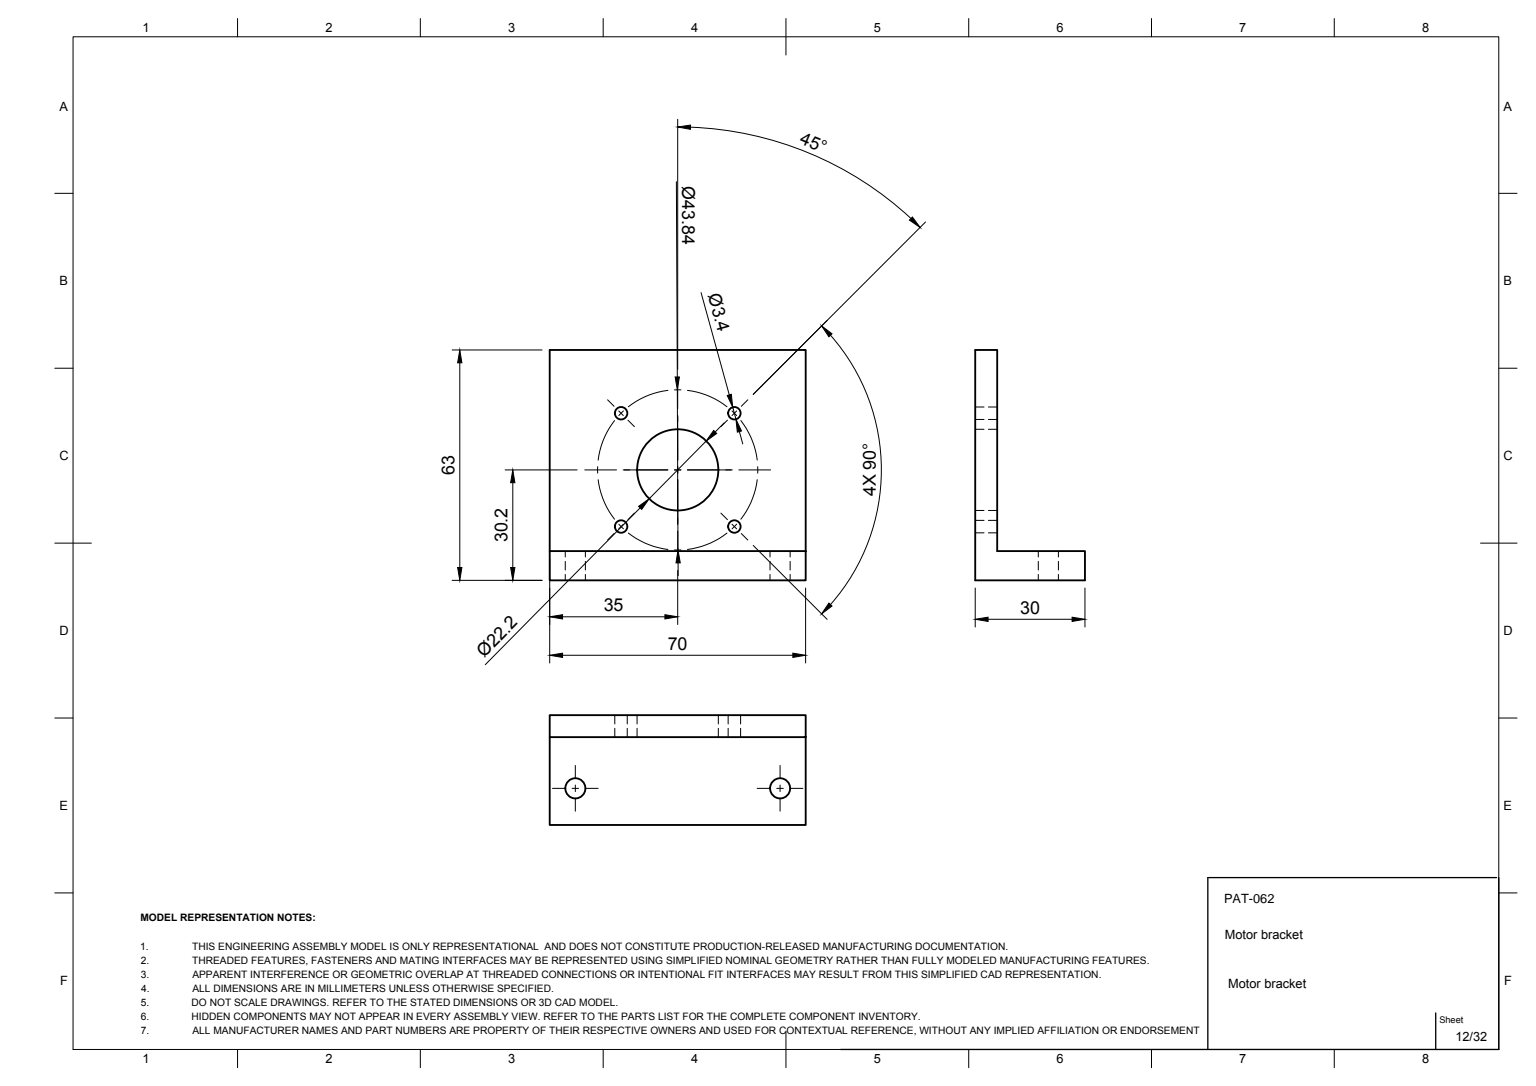
ISO-10303-21;
HEADER;
/* Generated by software containing ST-Developer
 * from STEP Tools, Inc. (www.steptools.com) 
 */

FILE_DESCRIPTION(
/* description */ ('Jaw-coupled motor to shaft test stand'),
/* implementation_level */ '2;1');

FILE_NAME(
/* name */ 'Motor bracket.step',
/* time_stamp */ '2026-10-27T10:46:06-07:00',
/* author */ (''),
/* organization */ (''),
/* preprocessor_version */ 'ST-DEVELOPER v20.2',
/* originating_system */ 'Autodesk Translation Framework v15.17.0.0',
/* authorisation */ '');

FILE_SCHEMA (('AUTOMOTIVE_DESIGN { 1 0 10303 214 3 1 1 }'));
ENDSEC;

DATA;
#10=MECHANICAL_DESIGN_GEOMETRIC_PRESENTATION_REPRESENTATION('',(#347),#19361);
#283=SHAPE_REPRESENTATION_RELATIONSHIP('SRR','None',#19497,#315);
#315=ADVANCED_BREP_SHAPE_REPRESENTATION('',(#380),#19333);
#347=STYLED_ITEM('',(#19725),#380);
#380=MANIFOLD_SOLID_BREP('Body1',#10991);
#423=FACE_BOUND('',#1710,.T.);
#424=FACE_BOUND('',#1711,.T.);
#425=FACE_BOUND('',#1714,.T.);
#426=FACE_BOUND('',#1715,.T.);
#427=FACE_BOUND('',#1716,.T.);
#428=FACE_BOUND('',#1717,.T.);
#429=FACE_BOUND('',#1718,.T.);
#430=FACE_BOUND('',#1722,.T.);
#431=FACE_BOUND('',#1723,.T.);
#432=FACE_BOUND('',#1724,.T.);
#433=FACE_BOUND('',#1725,.T.);
#434=FACE_BOUND('',#1726,.T.);
#435=FACE_BOUND('',#1729,.T.);
#436=FACE_BOUND('',#1730,.T.);
#542=PLANE('',#11472);
#543=PLANE('',#11473);
#544=PLANE('',#11474);
#545=PLANE('',#11475);
#546=PLANE('',#11476);
#547=PLANE('',#11477);
#548=PLANE('',#11478);
#549=PLANE('',#11479);
#1062=FACE_OUTER_BOUND('',#1702,.T.);
#1063=FACE_OUTER_BOUND('',#1703,.T.);
#1064=FACE_OUTER_BOUND('',#1704,.T.);
#1065=FACE_OUTER_BOUND('',#1705,.T.);
#1066=FACE_OUTER_BOUND('',#1706,.T.);
#1067=FACE_OUTER_BOUND('',#1707,.T.);
#1068=FACE_OUTER_BOUND('',#1708,.T.);
#1069=FACE_OUTER_BOUND('',#1709,.T.);
#1070=FACE_OUTER_BOUND('',#1712,.T.);
#1071=FACE_OUTER_BOUND('',#1713,.T.);
#1072=FACE_OUTER_BOUND('',#1719,.T.);
#1073=FACE_OUTER_BOUND('',#1720,.T.);
#1074=FACE_OUTER_BOUND('',#1721,.T.);
#1075=FACE_OUTER_BOUND('',#1727,.T.);
#1076=FACE_OUTER_BOUND('',#1728,.T.);
#1702=EDGE_LOOP('',(#7502,#7503,#7504,#7505));
#1703=EDGE_LOOP('',(#7506,#7507,#7508,#7509));
#1704=EDGE_LOOP('',(#7510,#7511,#7512,#7513));
#1705=EDGE_LOOP('',(#7514,#7515,#7516,#7517));
#1706=EDGE_LOOP('',(#7518,#7519,#7520,#7521));
#1707=EDGE_LOOP('',(#7522,#7523,#7524,#7525));
#1708=EDGE_LOOP('',(#7526,#7527,#7528,#7529));
#1709=EDGE_LOOP('',(#7530,#7531,#7532,#7533));
#1710=EDGE_LOOP('',(#7534));
#1711=EDGE_LOOP('',(#7535));
#1712=EDGE_LOOP('',(#7536,#7537,#7538,#7539));
#1713=EDGE_LOOP('',(#7540,#7541,#7542,#7543));
#1714=EDGE_LOOP('',(#7544));
#1715=EDGE_LOOP('',(#7545));
#1716=EDGE_LOOP('',(#7546));
#1717=EDGE_LOOP('',(#7547));
#1718=EDGE_LOOP('',(#7548));
#1719=EDGE_LOOP('',(#7549,#7550,#7551,#7552,#7553,#7554));
#1720=EDGE_LOOP('',(#7555,#7556,#7557,#7558,#7559,#7560));
#1721=EDGE_LOOP('',(#7561,#7562,#7563,#7564));
#1722=EDGE_LOOP('',(#7565));
#1723=EDGE_LOOP('',(#7566));
#1724=EDGE_LOOP('',(#7567));
#1725=EDGE_LOOP('',(#7568));
#1726=EDGE_LOOP('',(#7569));
#1727=EDGE_LOOP('',(#7570,#7571,#7572,#7573));
#1728=EDGE_LOOP('',(#7574,#7575,#7576,#7577));
#1729=EDGE_LOOP('',(#7578));
#1730=EDGE_LOOP('',(#7579));
#2425=LINE('',#15611,#3578);
#2426=LINE('',#15617,#3579);
#2427=LINE('',#15623,#3580);
#2428=LINE('',#15629,#3581);
#2429=LINE('',#15635,#3582);
#2430=LINE('',#15641,#3583);
#2431=LINE('',#15647,#3584);
#2432=LINE('',#15652,#3585);
#2433=LINE('',#15654,#3586);
#2434=LINE('',#15656,#3587);
#2435=LINE('',#15657,#3588);
#2436=LINE('',#15660,#3589);
#2437=LINE('',#15662,#3590);
#2438=LINE('',#15663,#3591);
#2439=LINE('',#15667,#3592);
#2440=LINE('',#15669,#3593);
#2441=LINE('',#15671,#3594);
#2442=LINE('',#15672,#3595);
#2443=LINE('',#15675,#3596);
#2444=LINE('',#15676,#3597);
#2445=LINE('',#15677,#3598);
#2446=LINE('',#15680,#3599);
#2447=LINE('',#15681,#3600);
#2448=LINE('',#15682,#3601);
#2449=LINE('',#15684,#3602);
#3578=VECTOR('',#12550,0.17);
#3579=VECTOR('',#12557,0.17);
#3580=VECTOR('',#12564,0.17);
#3581=VECTOR('',#12571,0.17);
#3582=VECTOR('',#12578,1.11);
#3583=VECTOR('',#12585,0.275);
#3584=VECTOR('',#12592,0.275);
#3585=VECTOR('',#12597,1.);
#3586=VECTOR('',#12598,1.);
#3587=VECTOR('',#12599,1.);
#3588=VECTOR('',#12600,1.);
#3589=VECTOR('',#12603,1.);
#3590=VECTOR('',#12604,1.);
#3591=VECTOR('',#12605,1.);
#3592=VECTOR('',#12608,1.);
#3593=VECTOR('',#12609,1.);
#3594=VECTOR('',#12610,1.);
#3595=VECTOR('',#12611,1.);
#3596=VECTOR('',#12614,1.);
#3597=VECTOR('',#12615,1.);
#3598=VECTOR('',#12616,1.);
#3599=VECTOR('',#12619,1.);
#3600=VECTOR('',#12620,1.);
#3601=VECTOR('',#12621,1.);
#3602=VECTOR('',#12624,1.);
#4709=CIRCLE('',#11452,0.17);
#4710=CIRCLE('',#11453,0.17);
#4711=CIRCLE('',#11455,0.17);
#4712=CIRCLE('',#11456,0.17);
#4713=CIRCLE('',#11458,0.17);
#4714=CIRCLE('',#11459,0.17);
#4715=CIRCLE('',#11461,0.17);
#4716=CIRCLE('',#11462,0.17);
#4717=CIRCLE('',#11464,1.11);
#4718=CIRCLE('',#11465,1.11);
#4719=CIRCLE('',#11467,0.275);
#4720=CIRCLE('',#11468,0.275);
#4721=CIRCLE('',#11470,0.275);
#4722=CIRCLE('',#11471,0.275);
#4995=VERTEX_POINT('',#15608);
#4996=VERTEX_POINT('',#15610);
#4997=VERTEX_POINT('',#15614);
#4998=VERTEX_POINT('',#15616);
#4999=VERTEX_POINT('',#15620);
#5000=VERTEX_POINT('',#15622);
#5001=VERTEX_POINT('',#15626);
#5002=VERTEX_POINT('',#15628);
#5003=VERTEX_POINT('',#15632);
#5004=VERTEX_POINT('',#15634);
#5005=VERTEX_POINT('',#15638);
#5006=VERTEX_POINT('',#15640);
#5007=VERTEX_POINT('',#15644);
#5008=VERTEX_POINT('',#15646);
#5009=VERTEX_POINT('',#15650);
#5010=VERTEX_POINT('',#15651);
#5011=VERTEX_POINT('',#15653);
#5012=VERTEX_POINT('',#15655);
#5013=VERTEX_POINT('',#15659);
#5014=VERTEX_POINT('',#15661);
#5015=VERTEX_POINT('',#15665);
#5016=VERTEX_POINT('',#15666);
#5017=VERTEX_POINT('',#15668);
#5018=VERTEX_POINT('',#15670);
#5019=VERTEX_POINT('',#15674);
#5020=VERTEX_POINT('',#15679);
#5962=EDGE_CURVE('',#4995,#4995,#4709,.T.);
#5963=EDGE_CURVE('',#4995,#4996,#2425,.T.);
#5964=EDGE_CURVE('',#4996,#4996,#4710,.T.);
#5965=EDGE_CURVE('',#4997,#4997,#4711,.T.);
#5966=EDGE_CURVE('',#4997,#4998,#2426,.T.);
#5967=EDGE_CURVE('',#4998,#4998,#4712,.T.);
#5968=EDGE_CURVE('',#4999,#4999,#4713,.T.);
#5969=EDGE_CURVE('',#4999,#5000,#2427,.T.);
#5970=EDGE_CURVE('',#5000,#5000,#4714,.T.);
#5971=EDGE_CURVE('',#5001,#5001,#4715,.T.);
#5972=EDGE_CURVE('',#5001,#5002,#2428,.T.);
#5973=EDGE_CURVE('',#5002,#5002,#4716,.T.);
#5974=EDGE_CURVE('',#5003,#5003,#4717,.T.);
#5975=EDGE_CURVE('',#5003,#5004,#2429,.T.);
#5976=EDGE_CURVE('',#5004,#5004,#4718,.T.);
#5977=EDGE_CURVE('',#5005,#5005,#4719,.T.);
#5978=EDGE_CURVE('',#5005,#5006,#2430,.T.);
#5979=EDGE_CURVE('',#5006,#5006,#4720,.T.);
#5980=EDGE_CURVE('',#5007,#5007,#4721,.T.);
#5981=EDGE_CURVE('',#5007,#5008,#2431,.T.);
#5982=EDGE_CURVE('',#5008,#5008,#4722,.T.);
#5983=EDGE_CURVE('',#5009,#5010,#2432,.T.);
#5984=EDGE_CURVE('',#5011,#5009,#2433,.T.);
#5985=EDGE_CURVE('',#5012,#5011,#2434,.T.);
#5986=EDGE_CURVE('',#5012,#5010,#2435,.T.);
#5987=EDGE_CURVE('',#5011,#5013,#2436,.T.);
#5988=EDGE_CURVE('',#5013,#5014,#2437,.T.);
#5989=EDGE_CURVE('',#5014,#5012,#2438,.T.);
#5990=EDGE_CURVE('',#5015,#5016,#2439,.T.);
#5991=EDGE_CURVE('',#5017,#5016,#2440,.T.);
#5992=EDGE_CURVE('',#5018,#5017,#2441,.T.);
#5993=EDGE_CURVE('',#5018,#5015,#2442,.T.);
#5994=EDGE_CURVE('',#5009,#5019,#2443,.T.);
#5995=EDGE_CURVE('',#5016,#5019,#2444,.T.);
#5996=EDGE_CURVE('',#5015,#5013,#2445,.T.);
#5997=EDGE_CURVE('',#5020,#5017,#2446,.T.);
#5998=EDGE_CURVE('',#5010,#5020,#2447,.T.);
#5999=EDGE_CURVE('',#5014,#5018,#2448,.T.);
#6000=EDGE_CURVE('',#5019,#5020,#2449,.T.);
#7502=ORIENTED_EDGE('',*,*,#5962,.F.);
#7503=ORIENTED_EDGE('',*,*,#5963,.T.);
#7504=ORIENTED_EDGE('',*,*,#5964,.F.);
#7505=ORIENTED_EDGE('',*,*,#5963,.F.);
#7506=ORIENTED_EDGE('',*,*,#5965,.F.);
#7507=ORIENTED_EDGE('',*,*,#5966,.T.);
#7508=ORIENTED_EDGE('',*,*,#5967,.F.);
#7509=ORIENTED_EDGE('',*,*,#5966,.F.);
#7510=ORIENTED_EDGE('',*,*,#5968,.F.);
#7511=ORIENTED_EDGE('',*,*,#5969,.T.);
#7512=ORIENTED_EDGE('',*,*,#5970,.F.);
#7513=ORIENTED_EDGE('',*,*,#5969,.F.);
#7514=ORIENTED_EDGE('',*,*,#5971,.F.);
#7515=ORIENTED_EDGE('',*,*,#5972,.T.);
#7516=ORIENTED_EDGE('',*,*,#5973,.F.);
#7517=ORIENTED_EDGE('',*,*,#5972,.F.);
#7518=ORIENTED_EDGE('',*,*,#5974,.F.);
#7519=ORIENTED_EDGE('',*,*,#5975,.T.);
#7520=ORIENTED_EDGE('',*,*,#5976,.F.);
#7521=ORIENTED_EDGE('',*,*,#5975,.F.);
#7522=ORIENTED_EDGE('',*,*,#5977,.F.);
#7523=ORIENTED_EDGE('',*,*,#5978,.T.);
#7524=ORIENTED_EDGE('',*,*,#5979,.F.);
#7525=ORIENTED_EDGE('',*,*,#5978,.F.);
#7526=ORIENTED_EDGE('',*,*,#5980,.F.);
#7527=ORIENTED_EDGE('',*,*,#5981,.T.);
#7528=ORIENTED_EDGE('',*,*,#5982,.F.);
#7529=ORIENTED_EDGE('',*,*,#5981,.F.);
#7530=ORIENTED_EDGE('',*,*,#5983,.F.);
#7531=ORIENTED_EDGE('',*,*,#5984,.F.);
#7532=ORIENTED_EDGE('',*,*,#5985,.F.);
#7533=ORIENTED_EDGE('',*,*,#5986,.T.);
#7534=ORIENTED_EDGE('',*,*,#5979,.T.);
#7535=ORIENTED_EDGE('',*,*,#5982,.T.);
#7536=ORIENTED_EDGE('',*,*,#5985,.T.);
#7537=ORIENTED_EDGE('',*,*,#5987,.T.);
#7538=ORIENTED_EDGE('',*,*,#5988,.T.);
#7539=ORIENTED_EDGE('',*,*,#5989,.T.);
#7540=ORIENTED_EDGE('',*,*,#5990,.T.);
#7541=ORIENTED_EDGE('',*,*,#5991,.F.);
#7542=ORIENTED_EDGE('',*,*,#5992,.F.);
#7543=ORIENTED_EDGE('',*,*,#5993,.T.);
#7544=ORIENTED_EDGE('',*,*,#5976,.T.);
#7545=ORIENTED_EDGE('',*,*,#5973,.T.);
#7546=ORIENTED_EDGE('',*,*,#5970,.T.);
#7547=ORIENTED_EDGE('',*,*,#5967,.T.);
#7548=ORIENTED_EDGE('',*,*,#5964,.T.);
#7549=ORIENTED_EDGE('',*,*,#5994,.T.);
#7550=ORIENTED_EDGE('',*,*,#5995,.F.);
#7551=ORIENTED_EDGE('',*,*,#5990,.F.);
#7552=ORIENTED_EDGE('',*,*,#5996,.T.);
#7553=ORIENTED_EDGE('',*,*,#5987,.F.);
#7554=ORIENTED_EDGE('',*,*,#5984,.T.);
#7555=ORIENTED_EDGE('',*,*,#5992,.T.);
#7556=ORIENTED_EDGE('',*,*,#5997,.F.);
#7557=ORIENTED_EDGE('',*,*,#5998,.F.);
#7558=ORIENTED_EDGE('',*,*,#5986,.F.);
#7559=ORIENTED_EDGE('',*,*,#5989,.F.);
#7560=ORIENTED_EDGE('',*,*,#5999,.T.);
#7561=ORIENTED_EDGE('',*,*,#5983,.T.);
#7562=ORIENTED_EDGE('',*,*,#5998,.T.);
#7563=ORIENTED_EDGE('',*,*,#6000,.F.);
#7564=ORIENTED_EDGE('',*,*,#5994,.F.);
#7565=ORIENTED_EDGE('',*,*,#5974,.T.);
#7566=ORIENTED_EDGE('',*,*,#5971,.T.);
#7567=ORIENTED_EDGE('',*,*,#5968,.T.);
#7568=ORIENTED_EDGE('',*,*,#5965,.T.);
#7569=ORIENTED_EDGE('',*,*,#5962,.T.);
#7570=ORIENTED_EDGE('',*,*,#5995,.T.);
#7571=ORIENTED_EDGE('',*,*,#6000,.T.);
#7572=ORIENTED_EDGE('',*,*,#5997,.T.);
#7573=ORIENTED_EDGE('',*,*,#5991,.T.);
#7574=ORIENTED_EDGE('',*,*,#5996,.F.);
#7575=ORIENTED_EDGE('',*,*,#5993,.F.);
#7576=ORIENTED_EDGE('',*,*,#5999,.F.);
#7577=ORIENTED_EDGE('',*,*,#5988,.F.);
#7578=ORIENTED_EDGE('',*,*,#5977,.T.);
#7579=ORIENTED_EDGE('',*,*,#5980,.T.);
#10284=CYLINDRICAL_SURFACE('',#11451,0.17);
#10285=CYLINDRICAL_SURFACE('',#11454,0.17);
#10286=CYLINDRICAL_SURFACE('',#11457,0.17);
#10287=CYLINDRICAL_SURFACE('',#11460,0.17);
#10288=CYLINDRICAL_SURFACE('',#11463,1.11);
#10289=CYLINDRICAL_SURFACE('',#11466,0.275);
#10290=CYLINDRICAL_SURFACE('',#11469,0.275);
#10404=ADVANCED_FACE('',(#1062),#10284,.F.);
#10405=ADVANCED_FACE('',(#1063),#10285,.F.);
#10406=ADVANCED_FACE('',(#1064),#10286,.F.);
#10407=ADVANCED_FACE('',(#1065),#10287,.F.);
#10408=ADVANCED_FACE('',(#1066),#10288,.F.);
#10409=ADVANCED_FACE('',(#1067),#10289,.F.);
#10410=ADVANCED_FACE('',(#1068),#10290,.F.);
#10411=ADVANCED_FACE('',(#1069,#423,#424),#542,.T.);
#10412=ADVANCED_FACE('',(#1070),#543,.F.);
#10413=ADVANCED_FACE('',(#1071,#425,#426,#427,#428,#429),#544,.T.);
#10414=ADVANCED_FACE('',(#1072),#545,.T.);
#10415=ADVANCED_FACE('',(#1073),#546,.T.);
#10416=ADVANCED_FACE('',(#1074,#430,#431,#432,#433,#434),#547,.T.);
#10417=ADVANCED_FACE('',(#1075),#548,.T.);
#10418=ADVANCED_FACE('',(#1076,#435,#436),#549,.F.);
#10991=CLOSED_SHELL('',(#10404,#10405,#10406,#10407,#10408,#10409,#10410,
#10411,#10412,#10413,#10414,#10415,#10416,#10417,#10418));
#11450=AXIS2_PLACEMENT_3D('',#15606,#12544,#12545);
#11451=AXIS2_PLACEMENT_3D('',#15607,#12546,#12547);
#11452=AXIS2_PLACEMENT_3D('',#15609,#12548,#12549);
#11453=AXIS2_PLACEMENT_3D('',#15612,#12551,#12552);
#11454=AXIS2_PLACEMENT_3D('',#15613,#12553,#12554);
#11455=AXIS2_PLACEMENT_3D('',#15615,#12555,#12556);
#11456=AXIS2_PLACEMENT_3D('',#15618,#12558,#12559);
#11457=AXIS2_PLACEMENT_3D('',#15619,#12560,#12561);
#11458=AXIS2_PLACEMENT_3D('',#15621,#12562,#12563);
#11459=AXIS2_PLACEMENT_3D('',#15624,#12565,#12566);
#11460=AXIS2_PLACEMENT_3D('',#15625,#12567,#12568);
#11461=AXIS2_PLACEMENT_3D('',#15627,#12569,#12570);
#11462=AXIS2_PLACEMENT_3D('',#15630,#12572,#12573);
#11463=AXIS2_PLACEMENT_3D('',#15631,#12574,#12575);
#11464=AXIS2_PLACEMENT_3D('',#15633,#12576,#12577);
#11465=AXIS2_PLACEMENT_3D('',#15636,#12579,#12580);
#11466=AXIS2_PLACEMENT_3D('',#15637,#12581,#12582);
#11467=AXIS2_PLACEMENT_3D('',#15639,#12583,#12584);
#11468=AXIS2_PLACEMENT_3D('',#15642,#12586,#12587);
#11469=AXIS2_PLACEMENT_3D('',#15643,#12588,#12589);
#11470=AXIS2_PLACEMENT_3D('',#15645,#12590,#12591);
#11471=AXIS2_PLACEMENT_3D('',#15648,#12593,#12594);
#11472=AXIS2_PLACEMENT_3D('',#15649,#12595,#12596);
#11473=AXIS2_PLACEMENT_3D('',#15658,#12601,#12602);
#11474=AXIS2_PLACEMENT_3D('',#15664,#12606,#12607);
#11475=AXIS2_PLACEMENT_3D('',#15673,#12612,#12613);
#11476=AXIS2_PLACEMENT_3D('',#15678,#12617,#12618);
#11477=AXIS2_PLACEMENT_3D('',#15683,#12622,#12623);
#11478=AXIS2_PLACEMENT_3D('',#15685,#12625,#12626);
#11479=AXIS2_PLACEMENT_3D('',#15686,#12627,#12628);
#12544=DIRECTION('axis',(0.,0.,1.));
#12545=DIRECTION('refdir',(1.,0.,0.));
#12546=DIRECTION('center_axis',(0.,1.,0.));
#12547=DIRECTION('ref_axis',(1.,0.,0.));
#12548=DIRECTION('center_axis',(0.,1.,0.));
#12549=DIRECTION('ref_axis',(1.,0.,0.));
#12550=DIRECTION('',(0.,1.,0.));
#12551=DIRECTION('center_axis',(0.,-1.,0.));
#12552=DIRECTION('ref_axis',(1.,0.,0.));
#12553=DIRECTION('center_axis',(0.,1.,0.));
#12554=DIRECTION('ref_axis',(1.,0.,0.));
#12555=DIRECTION('center_axis',(0.,1.,0.));
#12556=DIRECTION('ref_axis',(1.,0.,0.));
#12557=DIRECTION('',(0.,1.,0.));
#12558=DIRECTION('center_axis',(0.,-1.,0.));
#12559=DIRECTION('ref_axis',(1.,0.,0.));
#12560=DIRECTION('center_axis',(0.,1.,0.));
#12561=DIRECTION('ref_axis',(1.,0.,0.));
#12562=DIRECTION('center_axis',(0.,1.,0.));
#12563=DIRECTION('ref_axis',(1.,0.,0.));
#12564=DIRECTION('',(0.,1.,0.));
#12565=DIRECTION('center_axis',(0.,-1.,0.));
#12566=DIRECTION('ref_axis',(1.,0.,0.));
#12567=DIRECTION('center_axis',(0.,1.,0.));
#12568=DIRECTION('ref_axis',(1.,0.,0.));
#12569=DIRECTION('center_axis',(0.,1.,0.));
#12570=DIRECTION('ref_axis',(1.,0.,0.));
#12571=DIRECTION('',(0.,1.,0.));
#12572=DIRECTION('center_axis',(0.,-1.,0.));
#12573=DIRECTION('ref_axis',(1.,0.,0.));
#12574=DIRECTION('center_axis',(0.,1.,0.));
#12575=DIRECTION('ref_axis',(1.,0.,0.));
#12576=DIRECTION('center_axis',(0.,1.,0.));
#12577=DIRECTION('ref_axis',(1.,0.,0.));
#12578=DIRECTION('',(0.,1.,0.));
#12579=DIRECTION('center_axis',(0.,-1.,0.));
#12580=DIRECTION('ref_axis',(1.,0.,0.));
#12581=DIRECTION('center_axis',(0.,0.,1.));
#12582=DIRECTION('ref_axis',(1.,0.,0.));
#12583=DIRECTION('center_axis',(0.,0.,1.));
#12584=DIRECTION('ref_axis',(1.,0.,0.));
#12585=DIRECTION('',(0.,0.,1.));
#12586=DIRECTION('center_axis',(0.,0.,-1.));
#12587=DIRECTION('ref_axis',(1.,0.,0.));
#12588=DIRECTION('center_axis',(0.,0.,1.));
#12589=DIRECTION('ref_axis',(1.,0.,0.));
#12590=DIRECTION('center_axis',(0.,0.,1.));
#12591=DIRECTION('ref_axis',(1.,0.,0.));
#12592=DIRECTION('',(0.,0.,1.));
#12593=DIRECTION('center_axis',(0.,0.,-1.));
#12594=DIRECTION('ref_axis',(1.,0.,0.));
#12595=DIRECTION('center_axis',(0.,0.,1.));
#12596=DIRECTION('ref_axis',(1.,0.,0.));
#12597=DIRECTION('',(1.,0.,0.));
#12598=DIRECTION('',(0.,1.,0.));
#12599=DIRECTION('',(-1.,0.,0.));
#12600=DIRECTION('',(0.,1.,0.));
#12601=DIRECTION('center_axis',(0.,1.,0.));
#12602=DIRECTION('ref_axis',(1.,0.,0.));
#12603=DIRECTION('',(0.,0.,-1.));
#12604=DIRECTION('',(1.,0.,0.));
#12605=DIRECTION('',(0.,0.,1.));
#12606=DIRECTION('center_axis',(0.,1.,0.));
#12607=DIRECTION('ref_axis',(-1.,0.,0.));
#12608=DIRECTION('',(0.,0.,1.));
#12609=DIRECTION('',(-1.,0.,0.));
#12610=DIRECTION('',(0.,0.,1.));
#12611=DIRECTION('',(-1.,0.,0.));
#12612=DIRECTION('center_axis',(-1.,0.,0.));
#12613=DIRECTION('ref_axis',(0.,-1.,0.));
#12614=DIRECTION('',(0.,0.,1.));
#12615=DIRECTION('',(0.,-1.,0.));
#12616=DIRECTION('',(0.,-1.,0.));
#12617=DIRECTION('center_axis',(1.,0.,0.));
#12618=DIRECTION('ref_axis',(0.,1.,0.));
#12619=DIRECTION('',(0.,1.,0.));
#12620=DIRECTION('',(0.,0.,1.));
#12621=DIRECTION('',(0.,1.,0.));
#12622=DIRECTION('center_axis',(0.,-1.,0.));
#12623=DIRECTION('ref_axis',(1.,0.,0.));
#12624=DIRECTION('',(1.,0.,0.));
#12625=DIRECTION('center_axis',(0.,0.,1.));
#12626=DIRECTION('ref_axis',(1.,0.,0.));
#12627=DIRECTION('center_axis',(0.,0.,1.));
#12628=DIRECTION('ref_axis',(1.,0.,0.));
#15606=CARTESIAN_POINT('',(0.,0.,0.));
#15607=CARTESIAN_POINT('Origin',(1.55,-7.7,2.67));
#15608=CARTESIAN_POINT('',(1.38,-7.6,2.67));
#15609=CARTESIAN_POINT('Origin',(1.55,-7.6,2.67));
#15610=CARTESIAN_POINT('',(1.38,-7.,2.67));
#15611=CARTESIAN_POINT('',(1.38,-7.7,2.67));
#15612=CARTESIAN_POINT('Origin',(1.55,-7.,2.67));
#15613=CARTESIAN_POINT('Origin',(-1.55,-7.7,5.77));
#15614=CARTESIAN_POINT('',(-1.72,-7.6,5.77));
#15615=CARTESIAN_POINT('Origin',(-1.55,-7.6,5.77));
#15616=CARTESIAN_POINT('',(-1.72,-7.,5.77));
#15617=CARTESIAN_POINT('',(-1.72,-7.7,5.77));
#15618=CARTESIAN_POINT('Origin',(-1.55,-7.,5.77));
#15619=CARTESIAN_POINT('Origin',(-1.55,-7.7,2.67));
#15620=CARTESIAN_POINT('',(-1.72,-7.6,2.67));
#15621=CARTESIAN_POINT('Origin',(-1.55,-7.6,2.67));
#15622=CARTESIAN_POINT('',(-1.72,-7.,2.67));
#15623=CARTESIAN_POINT('',(-1.72,-7.7,2.67));
#15624=CARTESIAN_POINT('Origin',(-1.55,-7.,2.67));
#15625=CARTESIAN_POINT('Origin',(1.55,-7.7,5.77));
#15626=CARTESIAN_POINT('',(1.38,-7.6,5.77));
#15627=CARTESIAN_POINT('Origin',(1.55,-7.6,5.77));
#15628=CARTESIAN_POINT('',(1.38,-7.,5.77));
#15629=CARTESIAN_POINT('',(1.38,-7.7,5.77));
#15630=CARTESIAN_POINT('Origin',(1.55,-7.,5.77));
#15631=CARTESIAN_POINT('Origin',(0.,-7.7,4.22));
#15632=CARTESIAN_POINT('',(-1.11,-7.6,4.22));
#15633=CARTESIAN_POINT('Origin',(0.,-7.6,4.22));
#15634=CARTESIAN_POINT('',(-1.11,-7.,4.22));
#15635=CARTESIAN_POINT('',(-1.11,-7.7,4.22));
#15636=CARTESIAN_POINT('Origin',(0.,-7.,4.22));
#15637=CARTESIAN_POINT('Origin',(-2.8,-9.,1.1));
#15638=CARTESIAN_POINT('',(-3.075,-9.,1.2));
#15639=CARTESIAN_POINT('Origin',(-2.8,-9.,1.2));
#15640=CARTESIAN_POINT('',(-3.075,-9.,2.));
#15641=CARTESIAN_POINT('',(-3.075,-9.,1.1));
#15642=CARTESIAN_POINT('Origin',(-2.8,-9.,2.));
#15643=CARTESIAN_POINT('Origin',(2.8,-9.,1.1));
#15644=CARTESIAN_POINT('',(2.525,-9.,1.2));
#15645=CARTESIAN_POINT('Origin',(2.8,-9.,1.2));
#15646=CARTESIAN_POINT('',(2.525,-9.,2.));
#15647=CARTESIAN_POINT('',(2.525,-9.,1.1));
#15648=CARTESIAN_POINT('Origin',(2.8,-9.,2.));
#15649=CARTESIAN_POINT('Origin',(-3.5,-10.,2.));
#15650=CARTESIAN_POINT('',(-3.5,-7.6,2.));
#15651=CARTESIAN_POINT('',(3.5,-7.6,2.));
#15652=CARTESIAN_POINT('',(-3.5,-7.6,2.));
#15653=CARTESIAN_POINT('',(-3.5,-10.,2.));
#15654=CARTESIAN_POINT('',(-3.5,-10.,2.));
#15655=CARTESIAN_POINT('',(3.5,-10.,2.));
#15656=CARTESIAN_POINT('',(3.5,-10.,2.));
#15657=CARTESIAN_POINT('',(3.5,-10.,2.));
#15658=CARTESIAN_POINT('Origin',(0.,-10.,1.6));
#15659=CARTESIAN_POINT('',(-3.5,-10.,1.2));
#15660=CARTESIAN_POINT('',(-3.5,-10.,2.));
#15661=CARTESIAN_POINT('',(3.5,-10.,1.2));
#15662=CARTESIAN_POINT('',(-3.5,-10.,1.2));
#15663=CARTESIAN_POINT('',(3.5,-10.,1.2));
#15664=CARTESIAN_POINT('Origin',(3.5,-7.,1.2));
#15665=CARTESIAN_POINT('',(-3.5,-7.,1.2));
#15666=CARTESIAN_POINT('',(-3.5,-7.,7.5));
#15667=CARTESIAN_POINT('',(-3.5,-7.,1.2));
#15668=CARTESIAN_POINT('',(3.5,-7.,7.5));
#15669=CARTESIAN_POINT('',(3.5,-7.,7.5));
#15670=CARTESIAN_POINT('',(3.5,-7.,1.2));
#15671=CARTESIAN_POINT('',(3.5,-7.,1.2));
#15672=CARTESIAN_POINT('',(3.5,-7.,1.2));
#15673=CARTESIAN_POINT('Origin',(-3.5,-7.,1.2));
#15674=CARTESIAN_POINT('',(-3.5,-7.6,7.5));
#15675=CARTESIAN_POINT('',(-3.5,-7.6,1.2));
#15676=CARTESIAN_POINT('',(-3.5,-7.,7.5));
#15677=CARTESIAN_POINT('',(-3.5,-7.,1.2));
#15678=CARTESIAN_POINT('Origin',(3.5,-7.6,1.2));
#15679=CARTESIAN_POINT('',(3.5,-7.6,7.5));
#15680=CARTESIAN_POINT('',(3.5,-7.6,7.5));
#15681=CARTESIAN_POINT('',(3.5,-7.6,1.2));
#15682=CARTESIAN_POINT('',(3.5,-10.,1.2));
#15683=CARTESIAN_POINT('Origin',(-3.5,-7.6,1.2));
#15684=CARTESIAN_POINT('',(-3.5,-7.6,7.5));
#15685=CARTESIAN_POINT('Origin',(0.,-7.3,7.5));
#15686=CARTESIAN_POINT('Origin',(0.,-7.3,1.2));
#19295=UNCERTAINTY_MEASURE_WITH_UNIT(LENGTH_MEASURE(0.001),#19362,
'DISTANCE_ACCURACY_VALUE',
'Maximum model space distance between geometric entities at asserted c
onnectivities');
#19323=UNCERTAINTY_MEASURE_WITH_UNIT(LENGTH_MEASURE(0.001),#19362,
'DISTANCE_ACCURACY_VALUE',
'Maximum model space distance between geometric entities at asserted c
onnectivities');
#19333=(
GEOMETRIC_REPRESENTATION_CONTEXT(3)
GLOBAL_UNCERTAINTY_ASSIGNED_CONTEXT((#19295))
GLOBAL_UNIT_ASSIGNED_CONTEXT((#19362,#19364,#19365))
REPRESENTATION_CONTEXT('','3D')
);
#19361=(
GEOMETRIC_REPRESENTATION_CONTEXT(3)
GLOBAL_UNCERTAINTY_ASSIGNED_CONTEXT((#19323))
GLOBAL_UNIT_ASSIGNED_CONTEXT((#19362,#19364,#19365))
REPRESENTATION_CONTEXT('','3D')
);
#19362=(
LENGTH_UNIT()
NAMED_UNIT(*)
SI_UNIT(.CENTI.,.METRE.)
);
#19364=(
NAMED_UNIT(*)
PLANE_ANGLE_UNIT()
SI_UNIT($,.RADIAN.)
);
#19365=(
NAMED_UNIT(*)
SI_UNIT($,.STERADIAN.)
SOLID_ANGLE_UNIT()
);
#19375=SHAPE_DEFINITION_REPRESENTATION(#19412,#19497);
#19412=PRODUCT_DEFINITION_SHAPE('',$,#19535);
#19497=SHAPE_REPRESENTATION('',(#11450),#19333);
#19525=PRODUCT_DEFINITION_CONTEXT('part definition',#19638,'design');
#19535=PRODUCT_DEFINITION('Motor bracket','Motor bracket',#19572,#19525);
#19572=PRODUCT_DEFINITION_FORMATION('',$,#19649);
#19638=APPLICATION_CONTEXT(
'Core Data for Automotive Mechanical Design Process');
#19639=PRODUCT_CONTEXT('part definition',#19638,'mechanical');
#19649=PRODUCT('Motor bracket','Motor bracket','Motor bracket',(#19639));
#19719=COLOUR_RGB('Dark Blue',0.08,0.2,0.34);
#19720=FILL_AREA_STYLE_COLOUR('',#19719);
#19721=FILL_AREA_STYLE('',(#19720));
#19722=SURFACE_STYLE_FILL_AREA(#19721);
#19723=SURFACE_SIDE_STYLE('',(#19722));
#19724=SURFACE_STYLE_USAGE(.BOTH.,#19723);
#19725=PRESENTATION_STYLE_ASSIGNMENT((#19724));
ENDSEC;
END-ISO-10303-21;
